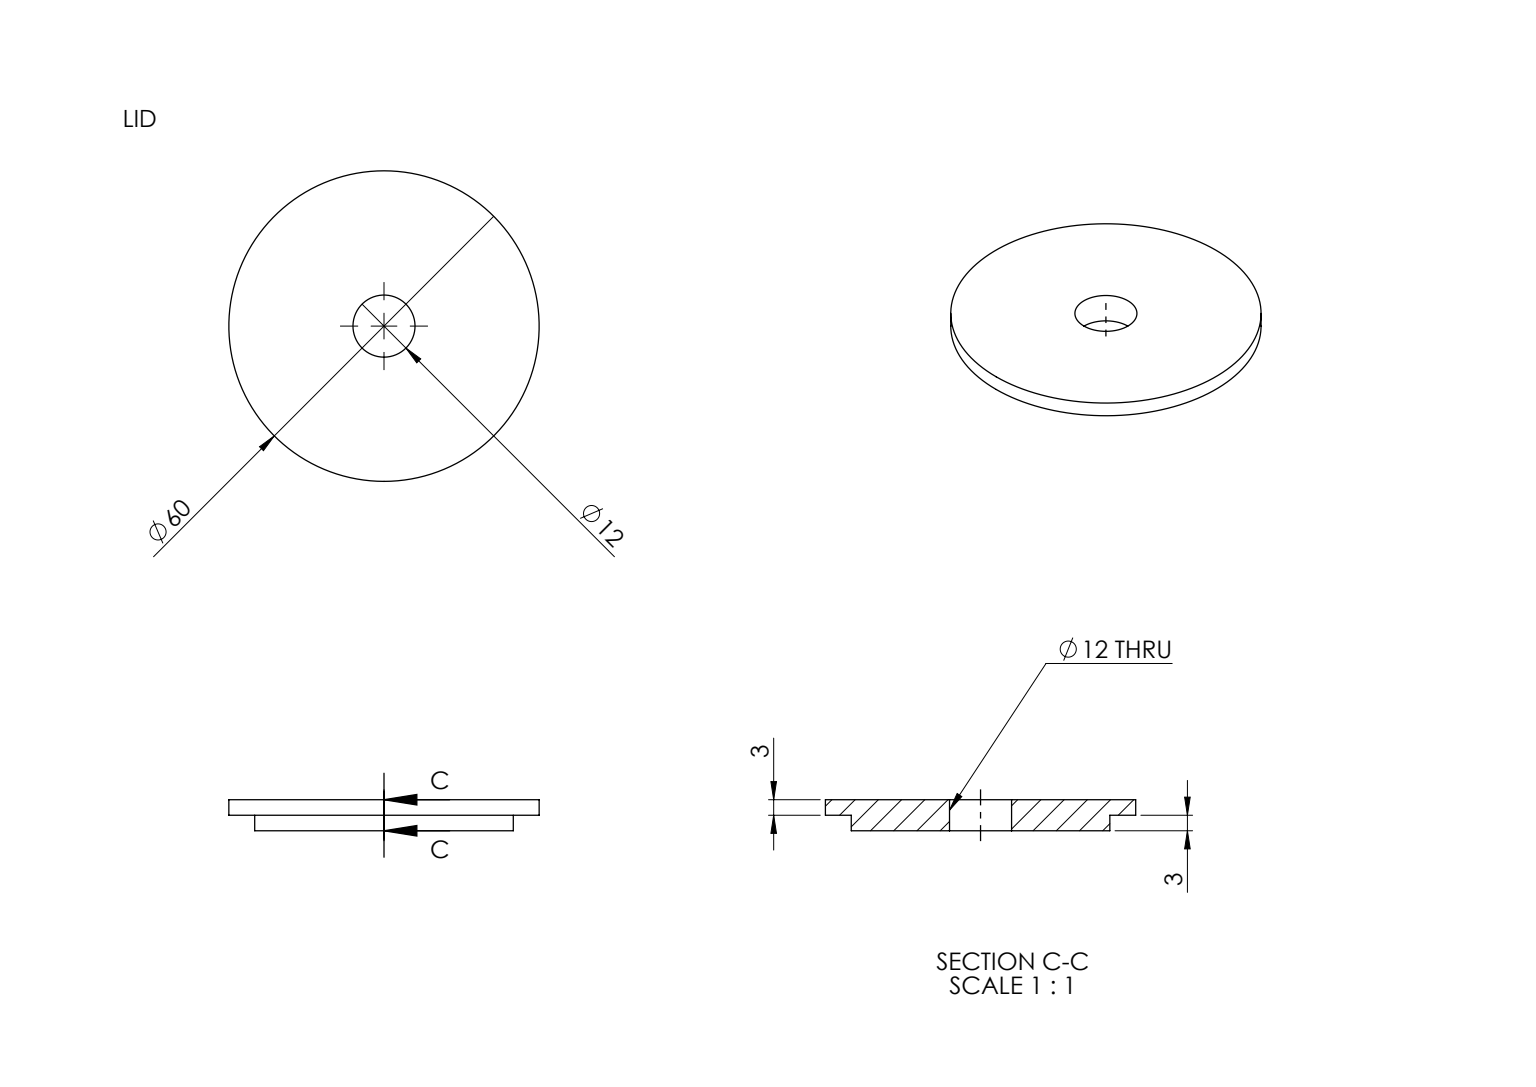
ISO-10303-21;
HEADER;
FILE_DESCRIPTION (('STEP AP214'),
    '1' );
FILE_NAME ('lid.step',
    '2026-10-04T07:23:31',
    ( '' ),
    ( '' ),
    'SwSTEP 2.0',
    'SolidWorks 2026',
    '' );
FILE_SCHEMA (( 'AUTOMOTIVE_DESIGN' ));
ENDSEC;

DATA;
#32=ADVANCED_FACE ( 'NONE', ( #4472 ), #1742, .F. ) ;
#73=CARTESIAN_POINT ( 'NONE',  ( 7.347880794884120722E-16, 82.00000000000000000, -6.000000000000000888 ) ) ;
#113=( NAMED_UNIT ( * ) SI_UNIT ( $, .STERADIAN. ) SOLID_ANGLE_UNIT ( ) );
#161=CARTESIAN_POINT ( 'NONE',  ( 0.000000000000000000, 85.00000000000000000, 0.000000000000000000 ) ) ;
#171=( LENGTH_UNIT ( ) NAMED_UNIT ( * ) SI_UNIT ( .MILLI., .METRE. ) );
#236=VECTOR ( 'NONE', #2762, 1000.000000000000000 ) ;
#246=LINE ( 'NONE', #73, #236 ) ;
#346=VERTEX_POINT ( 'NONE', #9726 ) ;
#355=DIRECTION ( 'NONE',  ( 0.000000000000000000, 1.000000000000000000, 0.000000000000000000 ) ) ;
#357=VECTOR ( 'NONE', #4991, 1000.000000000000000 ) ;
#379=CARTESIAN_POINT ( 'NONE',  ( 0.000000000000000000, 82.00000000000000000, 25.00000000000000000 ) ) ;
#411=FACE_OUTER_BOUND ( 'NONE', #2991, .T. ) ;
#443=EDGE_LOOP ( 'NONE', ( #4090, #2708 ) ) ;
#541=FILL_AREA_STYLE_COLOUR ( '', #3347 ) ;
#542=CARTESIAN_POINT ( 'NONE',  ( 3.061616997868383043E-15, 85.00000000000000000, -25.00000000000000000 ) ) ;
#599=( NAMED_UNIT ( * ) PLANE_ANGLE_UNIT ( ) SI_UNIT ( $, .RADIAN. ) );
#645=EDGE_LOOP ( 'NONE', ( #3984, #3500, #6506, #4878 ) ) ;
#724=LINE ( 'NONE', #5809, #357 ) ;
#759=AXIS2_PLACEMENT_3D ( 'NONE', #1982, #9602, #6241 ) ;
#766=CARTESIAN_POINT ( 'NONE',  ( 0.000000000000000000, 82.00000000000000000, 0.000000000000000000 ) ) ;
#786=CARTESIAN_POINT ( 'NONE',  ( 0.000000000000000000, 82.00000000000000000, 0.000000000000000000 ) ) ;
#791=EDGE_CURVE ( 'NONE', #2046, #346, #7043, .T. ) ;
#911=LINE ( 'NONE', #7643, #8108 ) ;
#959=CYLINDRICAL_SURFACE ( 'NONE', #3390, 6.000000000000000888 ) ;
#1022=DIRECTION ( 'NONE',  ( 0.000000000000000000, 1.000000000000000000, 0.000000000000000000 ) ) ;
#1025=DIRECTION ( 'NONE',  ( 0.000000000000000000, 0.000000000000000000, 1.000000000000000000 ) ) ;
#1035=DIRECTION ( 'NONE',  ( 0.000000000000000000, 1.000000000000000000, 0.000000000000000000 ) ) ;
#1113=FACE_OUTER_BOUND ( 'NONE', #1896, .T. ) ;
#1171=PLANE ( 'NONE',  #8884 ) ;
#1238=CARTESIAN_POINT ( 'NONE',  ( 0.000000000000000000, 82.00000000000000000, 0.000000000000000000 ) ) ;
#1280=( NAMED_UNIT ( * ) SI_UNIT ( $, .STERADIAN. ) SOLID_ANGLE_UNIT ( ) );
#1293=ORIENTED_EDGE ( 'NONE', *, *, #10193, .F. ) ;
#1298=PLANE ( 'NONE',  #6558 ) ;
#1332=PRODUCT ( 'lid', 'lid', '', ( #9152 ) ) ;
#1346=ORIENTED_EDGE ( 'NONE', *, *, #6014, .T. ) ;
#1382=DIRECTION ( 'NONE',  ( 0.000000000000000000, 1.000000000000000000, 0.000000000000000000 ) ) ;
#1465=CIRCLE ( 'NONE', #6577, 30.00000000000000000 ) ;
#1582=DIRECTION ( 'NONE',  ( 0.000000000000000000, 1.000000000000000000, 0.000000000000000000 ) ) ;
#1595=MECHANICAL_DESIGN_GEOMETRIC_PRESENTATION_REPRESENTATION('',(#7787),#10427);
#1619=CIRCLE ( 'NONE', #8151, 6.000000000000000888 ) ;
#1658=VERTEX_POINT ( 'NONE', #7012 ) ;
#1667=DIRECTION ( 'NONE',  ( 0.000000000000000000, 0.000000000000000000, 1.000000000000000000 ) ) ;
#1728=DIRECTION ( 'NONE',  ( 0.000000000000000000, 0.000000000000000000, 1.000000000000000000 ) ) ;
#1742=CYLINDRICAL_SURFACE ( 'NONE', #7907, 6.000000000000000888 ) ;
#1896=EDGE_LOOP ( 'NONE', ( #9721, #7390 ) ) ;
#1904=CARTESIAN_POINT ( 'NONE',  ( 0.000000000000000000, 0.000000000000000000, 0.000000000000000000 ) ) ;
#1945=LINE ( 'NONE', #3530, #6745 ) ;
#1982=CARTESIAN_POINT ( 'NONE',  ( 0.000000000000000000, 85.00000000000000000, 0.000000000000000000 ) ) ;
#2046=VERTEX_POINT ( 'NONE', #3882 ) ;
#2085=AXIS2_PLACEMENT_3D ( 'NONE', #5285, #6996, #1025 ) ;
#2090=ORIENTED_EDGE ( 'NONE', *, *, #10525, .T. ) ;
#2190=CARTESIAN_POINT ( 'NONE',  ( 0.000000000000000000, 88.00000000000001421, 0.000000000000000000 ) ) ;
#2227=ORIENTED_EDGE ( 'NONE', *, *, #4533, .T. ) ;
#2448=DIRECTION ( 'NONE',  ( 0.000000000000000000, -0.000000000000000000, 1.000000000000000000 ) ) ;
#2451=EDGE_CURVE ( 'NONE', #4148, #1658, #724, .T. ) ;
#2496=EDGE_LOOP ( 'NONE', ( #4124, #10919, #4863, #5660 ) ) ;
#2571=EDGE_CURVE ( 'NONE', #2830, #6236, #911, .T. ) ;
#2654=ORIENTED_EDGE ( 'NONE', *, *, #2571, .F. ) ;
#2708=ORIENTED_EDGE ( 'NONE', *, *, #10525, .F. ) ;
#2729=DIRECTION ( 'NONE',  ( 0.000000000000000000, 0.000000000000000000, 1.000000000000000000 ) ) ;
#2762=DIRECTION ( 'NONE',  ( 0.000000000000000000, 1.000000000000000000, 0.000000000000000000 ) ) ;
#2796=CARTESIAN_POINT ( 'NONE',  ( 0.000000000000000000, 85.00000000000000000, 0.000000000000000000 ) ) ;
#2821=CARTESIAN_POINT ( 'NONE',  ( 0.000000000000000000, 88.00000000000001421, 0.000000000000000000 ) ) ;
#2830=VERTEX_POINT ( 'NONE', #9435 ) ;
#2833=VECTOR ( 'NONE', #4440, 1000.000000000000000 ) ;
#2964=ORIENTED_EDGE ( 'NONE', *, *, #7197, .T. ) ;
#2984=EDGE_CURVE ( 'NONE', #6236, #1658, #4434, .T. ) ;
#2991=EDGE_LOOP ( 'NONE', ( #6706, #7409 ) ) ;
#3041=UNCERTAINTY_MEASURE_WITH_UNIT (LENGTH_MEASURE( 1.000000000000000082E-05 ), #5577, 'distance_accuracy_value', 'NONE');
#3072=SURFACE_STYLE_FILL_AREA ( #5529 ) ;
#3103=FACE_OUTER_BOUND ( 'NONE', #5298, .T. ) ;
#3222=SURFACE_SIDE_STYLE ('',( #10822 ) ) ;
#3230=VERTEX_POINT ( 'NONE', #10545 ) ;
#3247=EDGE_CURVE ( 'NONE', #7302, #6283, #9549, .T. ) ;
#3256=FACE_OUTER_BOUND ( 'NONE', #2496, .T. ) ;
#3276=DIRECTION ( 'NONE',  ( 0.000000000000000000, 0.000000000000000000, 1.000000000000000000 ) ) ;
#3290=CARTESIAN_POINT ( 'NONE',  ( 0.000000000000000000, 85.00000000000000000, 0.000000000000000000 ) ) ;
#3337=AXIS2_PLACEMENT_3D ( 'NONE', #3290, #1382, #4824 ) ;
#3347=COLOUR_RGB ( '', 0.66274510, 0.83137255, 0.94901961) ;
#3360=MANIFOLD_SOLID_BREP ( 'Boss-Extrude2', #5953 ) ;
#3390=AXIS2_PLACEMENT_3D ( 'NONE', #786, #7684, #1667 ) ;
#3428=DIRECTION ( 'NONE',  ( 0.000000000000000000, 1.000000000000000000, 0.000000000000000000 ) ) ;
#3431=DIRECTION ( 'NONE',  ( 0.000000000000000000, 0.000000000000000000, 1.000000000000000000 ) ) ;
#3473=CARTESIAN_POINT ( 'NONE',  ( 0.000000000000000000, 88.00000000000001421, 0.000000000000000000 ) ) ;
#3500=ORIENTED_EDGE ( 'NONE', *, *, #6344, .T. ) ;
#3503=ORIENTED_EDGE ( 'NONE', *, *, #3247, .F. ) ;
#3530=CARTESIAN_POINT ( 'NONE',  ( 3.061616997868383043E-15, 82.00000000000000000, -25.00000000000000000 ) ) ;
#3709=SURFACE_SIDE_STYLE ('',( #3072 ) ) ;
#3757=EDGE_CURVE ( 'NONE', #3230, #4608, #10227, .T. ) ;
#3793=CARTESIAN_POINT ( 'NONE',  ( 0.000000000000000000, 85.00000000000000000, 0.000000000000000000 ) ) ;
#3812=SURFACE_STYLE_USAGE ( .BOTH. , #3709 ) ;
#3882=CARTESIAN_POINT ( 'NONE',  ( 3.061616997868383043E-15, 82.00000000000000000, -25.00000000000000000 ) ) ;
#3888=ORIENTED_EDGE ( 'NONE', *, *, #10193, .T. ) ;
#3903=EDGE_CURVE ( 'NONE', #6283, #3230, #5920, .T. ) ;
#3953=UNCERTAINTY_MEASURE_WITH_UNIT (LENGTH_MEASURE( 1.000000000000000082E-05 ), #171, 'distance_accuracy_value', 'NONE');
#3961=VERTEX_POINT ( 'NONE', #7229 ) ;
#3984=ORIENTED_EDGE ( 'NONE', *, *, #10172, .T. ) ;
#4082=AXIS2_PLACEMENT_3D ( 'NONE', #9184, #9905, #4952 ) ;
#4090=ORIENTED_EDGE ( 'NONE', *, *, #3757, .F. ) ;
#4113=CIRCLE ( 'NONE', #5518, 25.00000000000000000 ) ;
#4124=ORIENTED_EDGE ( 'NONE', *, *, #6344, .F. ) ;
#4125=AXIS2_PLACEMENT_3D ( 'NONE', #6667, #10026, #2448 ) ;
#4131=AXIS2_PLACEMENT_3D ( 'NONE', #3793, #7165, #2729 ) ;
#4132=FACE_BOUND ( 'NONE', #443, .T. ) ;
#4148=VERTEX_POINT ( 'NONE', #6512 ) ;
#4155=DIRECTION ( 'NONE',  ( 0.000000000000000000, 1.000000000000000000, 0.000000000000000000 ) ) ;
#4204=FACE_OUTER_BOUND ( 'NONE', #4707, .T. ) ;
#4368=MECHANICAL_DESIGN_GEOMETRIC_PRESENTATION_REPRESENTATION('',(#10889),#10535);
#4418=PRODUCT_DEFINITION_FORMATION_WITH_SPECIFIED_SOURCE ( 'ANY', '', #1332, .NOT_KNOWN. ) ;
#4434=CIRCLE ( 'NONE', #3337, 30.00000000000000000 ) ;
#4440=DIRECTION ( 'NONE',  ( 0.000000000000000000, 1.000000000000000000, 0.000000000000000000 ) ) ;
#4472=FACE_OUTER_BOUND ( 'NONE', #10773, .T. ) ;
#4496=DIRECTION ( 'NONE',  ( 0.000000000000000000, 1.000000000000000000, 0.000000000000000000 ) ) ;
#4533=EDGE_CURVE ( 'NONE', #3961, #10543, #9708, .T. ) ;
#4572=DIRECTION ( 'NONE',  ( 0.000000000000000000, 0.000000000000000000, 1.000000000000000000 ) ) ;
#4585=FACE_OUTER_BOUND ( 'NONE', #9652, .T. ) ;
#4608=VERTEX_POINT ( 'NONE', #9501 ) ;
#4645=DIRECTION ( 'NONE',  ( 0.000000000000000000, 1.000000000000000000, 0.000000000000000000 ) ) ;
#4662=PRESENTATION_STYLE_ASSIGNMENT (( #3812 ) ) ;
#4707=EDGE_LOOP ( 'NONE', ( #3503, #3888, #2090, #5456 ) ) ;
#4779=ORIENTED_EDGE ( 'NONE', *, *, #2571, .T. ) ;
#4824=DIRECTION ( 'NONE',  ( 0.000000000000000000, 0.000000000000000000, 1.000000000000000000 ) ) ;
#4863=ORIENTED_EDGE ( 'NONE', *, *, #7668, .T. ) ;
#4878=ORIENTED_EDGE ( 'NONE', *, *, #7668, .F. ) ;
#4905=ADVANCED_FACE ( 'NONE', ( #9430, #4132 ), #8592, .T. ) ;
#4916=SHAPE_DEFINITION_REPRESENTATION ( #6369, #7685 ) ;
#4952=DIRECTION ( 'NONE',  ( 0.000000000000000000, 0.000000000000000000, 1.000000000000000000 ) ) ;
#4991=DIRECTION ( 'NONE',  ( -0.000000000000000000, -1.000000000000000000, -0.000000000000000000 ) ) ;
#5007=ADVANCED_FACE ( 'NONE', ( #4585 ), #6960, .T. ) ;
#5022=AXIS2_PLACEMENT_3D ( 'NONE', #7933, #9542, #8809 ) ;
#5051=EDGE_CURVE ( 'NONE', #10543, #3961, #10831, .T. ) ;
#5063=CYLINDRICAL_SURFACE ( 'NONE', #4082, 25.00000000000000000 ) ;
#5104=DIRECTION ( 'NONE',  ( 0.000000000000000000, 0.000000000000000000, 1.000000000000000000 ) ) ;
#5152=CARTESIAN_POINT ( 'NONE',  ( 0.000000000000000000, 85.00000000000000000, -30.00000000000000000 ) ) ;
#5285=CARTESIAN_POINT ( 'NONE',  ( 0.000000000000000000, 82.00000000000000000, 0.000000000000000000 ) ) ;
#5298=EDGE_LOOP ( 'NONE', ( #10761, #10694, #1346, #2654 ) ) ;
#5372=DIRECTION ( 'NONE',  ( 0.000000000000000000, 1.000000000000000000, 0.000000000000000000 ) ) ;
#5417=FACE_BOUND ( 'NONE', #5943, .T. ) ;
#5421=ORIENTED_EDGE ( 'NONE', *, *, #3757, .T. ) ;
#5440=FACE_BOUND ( 'NONE', #8351, .T. ) ;
#5456=ORIENTED_EDGE ( 'NONE', *, *, #3903, .F. ) ;
#5518=AXIS2_PLACEMENT_3D ( 'NONE', #7814, #1022, #1728 ) ;
#5529=FILL_AREA_STYLE ('',( #10550 ) ) ;
#5548=DIRECTION ( 'NONE',  ( 0.000000000000000000, 1.000000000000000000, 0.000000000000000000 ) ) ;
#5568=DIRECTION ( 'NONE',  ( -0.000000000000000000, -1.000000000000000000, -0.000000000000000000 ) ) ;
#5577=( LENGTH_UNIT ( ) NAMED_UNIT ( * ) SI_UNIT ( .MILLI., .METRE. ) );
#5653=DIRECTION ( 'NONE',  ( 0.000000000000000000, -0.000000000000000000, 1.000000000000000000 ) ) ;
#5660=ORIENTED_EDGE ( 'NONE', *, *, #5051, .F. ) ;
#5675=CYLINDRICAL_SURFACE ( 'NONE', #8858, 30.00000000000000000 ) ;
#5809=CARTESIAN_POINT ( 'NONE',  ( 3.673940397442059178E-15, 88.00000000000001421, 30.00000000000000000 ) ) ;
#5876=ORIENTED_EDGE ( 'NONE', *, *, #10242, .T. ) ;
#5877=CIRCLE ( 'NONE', #8705, 30.00000000000000000 ) ;
#5920=LINE ( 'NONE', #8621, #2833 ) ;
#5943=EDGE_LOOP ( 'NONE', ( #2227, #10087 ) ) ;
#5953=CLOSED_SHELL ( 'NONE', ( #6598, #7172, #10910, #8544, #8762, #32, #4905, #7690, #5007 ) ) ;
#5967=ORIENTED_EDGE ( 'NONE', *, *, #2451, .F. ) ;
#6014=EDGE_CURVE ( 'NONE', #1658, #6236, #10302, .T. ) ;
#6236=VERTEX_POINT ( 'NONE', #5152 ) ;
#6241=DIRECTION ( 'NONE',  ( 0.000000000000000000, 0.000000000000000000, 1.000000000000000000 ) ) ;
#6283=VERTEX_POINT ( 'NONE', #7799 ) ;
#6308=COLOUR_RGB ( '', 0.66274510, 0.83137255, 0.94901961) ;
#6344=EDGE_CURVE ( 'NONE', #2046, #10543, #1945, .T. ) ;
#6369=PRODUCT_DEFINITION_SHAPE ( 'NONE', 'NONE',  #8124 ) ;
#6411=EDGE_CURVE ( 'NONE', #6283, #7302, #1619, .T. ) ;
#6432=EDGE_LOOP ( 'NONE', ( #2964, #5876 ) ) ;
#6506=ORIENTED_EDGE ( 'NONE', *, *, #4533, .F. ) ;
#6512=CARTESIAN_POINT ( 'NONE',  ( 3.673940397442059178E-15, 88.00000000000001421, 30.00000000000000000 ) ) ;
#6558=AXIS2_PLACEMENT_3D ( 'NONE', #7155, #355, #5653 ) ;
#6577=AXIS2_PLACEMENT_3D ( 'NONE', #3473, #4155, #8345 ) ;
#6598=ADVANCED_FACE ( 'NONE', ( #3103 ), #5675, .T. ) ;
#6619=SURFACE_STYLE_USAGE ( .BOTH. , #3222 ) ;
#6667=CARTESIAN_POINT ( 'NONE',  ( 0.000000000000000000, 88.00000000000001421, 0.000000000000000000 ) ) ;
#6706=ORIENTED_EDGE ( 'NONE', *, *, #10172, .F. ) ;
#6745=VECTOR ( 'NONE', #9512, 1000.000000000000000 ) ;
#6893=DIRECTION ( 'NONE',  ( 0.000000000000000000, 0.000000000000000000, 1.000000000000000000 ) ) ;
#6908=ORIENTED_EDGE ( 'NONE', *, *, #6411, .F. ) ;
#6960=CYLINDRICAL_SURFACE ( 'NONE', #5022, 30.00000000000000000 ) ;
#6996=DIRECTION ( 'NONE',  ( 0.000000000000000000, 1.000000000000000000, 0.000000000000000000 ) ) ;
#7012=CARTESIAN_POINT ( 'NONE',  ( 3.673940397442059178E-15, 85.00000000000000000, 30.00000000000000000 ) ) ;
#7026=( GEOMETRIC_REPRESENTATION_CONTEXT ( 3 ) GLOBAL_UNCERTAINTY_ASSIGNED_CONTEXT ( ( #3953 ) ) GLOBAL_UNIT_ASSIGNED_CONTEXT ( ( #171, #9327, #113 ) ) REPRESENTATION_CONTEXT ( 'NONE', 'WORKASPACE' ) );
#7040=AXIS2_PLACEMENT_3D ( 'NONE', #1904, #3431, #7048 ) ;
#7043=CIRCLE ( 'NONE', #8242, 25.00000000000000000 ) ;
#7048=DIRECTION ( 'NONE',  ( 1.000000000000000000, 0.000000000000000000, 0.000000000000000000 ) ) ;
#7137=DIRECTION ( 'NONE',  ( 0.000000000000000000, 0.000000000000000000, 1.000000000000000000 ) ) ;
#7155=CARTESIAN_POINT ( 'NONE',  ( 0.000000000000000000, 82.00000000000000000, 0.000000000000000000 ) ) ;
#7165=DIRECTION ( 'NONE',  ( 0.000000000000000000, 1.000000000000000000, 0.000000000000000000 ) ) ;
#7172=ADVANCED_FACE ( 'NONE', ( #4204 ), #959, .F. ) ;
#7185=( NAMED_UNIT ( * ) PLANE_ANGLE_UNIT ( ) SI_UNIT ( $, .RADIAN. ) );
#7186=CARTESIAN_POINT ( 'NONE',  ( 7.347880794884120722E-16, 82.00000000000000000, -6.000000000000000888 ) ) ;
#7197=EDGE_CURVE ( 'NONE', #2830, #4148, #1465, .T. ) ;
#7229=CARTESIAN_POINT ( 'NONE',  ( 0.000000000000000000, 85.00000000000000000, 25.00000000000000000 ) ) ;
#7278=( NAMED_UNIT ( * ) SI_UNIT ( $, .STERADIAN. ) SOLID_ANGLE_UNIT ( ) );
#7298=DIRECTION ( 'NONE',  ( 0.000000000000000000, 1.000000000000000000, 0.000000000000000000 ) ) ;
#7302=VERTEX_POINT ( 'NONE', #7186 ) ;
#7316=DIRECTION ( 'NONE',  ( 0.000000000000000000, 0.000000000000000000, -1.000000000000000000 ) ) ;
#7390=ORIENTED_EDGE ( 'NONE', *, *, #6014, .F. ) ;
#7399=DIRECTION ( 'NONE',  ( 0.000000000000000000, 0.000000000000000000, 1.000000000000000000 ) ) ;
#7409=ORIENTED_EDGE ( 'NONE', *, *, #791, .F. ) ;
#7418=DIRECTION ( 'NONE',  ( -0.000000000000000000, -1.000000000000000000, -0.000000000000000000 ) ) ;
#7435=DIRECTION ( 'NONE',  ( 0.000000000000000000, 0.000000000000000000, 1.000000000000000000 ) ) ;
#7470=ORIENTED_EDGE ( 'NONE', *, *, #3247, .T. ) ;
#7499=CARTESIAN_POINT ( 'NONE',  ( 0.000000000000000000, 88.00000000000001421, 0.000000000000000000 ) ) ;
#7504=LINE ( 'NONE', #379, #7834 ) ;
#7538=CIRCLE ( 'NONE', #10003, 6.000000000000000888 ) ;
#7643=CARTESIAN_POINT ( 'NONE',  ( 0.000000000000000000, 88.00000000000001421, -30.00000000000000000 ) ) ;
#7652=CARTESIAN_POINT ( 'NONE',  ( 0.000000000000000000, 82.00000000000000000, 0.000000000000000000 ) ) ;
#7668=EDGE_CURVE ( 'NONE', #346, #3961, #7504, .T. ) ;
#7684=DIRECTION ( 'NONE',  ( 0.000000000000000000, 1.000000000000000000, 0.000000000000000000 ) ) ;
#7685=SHAPE_REPRESENTATION ( 'lid', ( #7040 ), #7026 ) ;
#7690=ADVANCED_FACE ( 'NONE', ( #5417, #1113 ), #1171, .F. ) ;
#7771=AXIS2_PLACEMENT_3D ( 'NONE', #2796, #4645, #10435 ) ;
#7787=STYLED_ITEM ( 'NONE', ( #10600 ), #3360 ) ;
#7799=CARTESIAN_POINT ( 'NONE',  ( 0.000000000000000000, 82.00000000000000000, 6.000000000000000888 ) ) ;
#7814=CARTESIAN_POINT ( 'NONE',  ( 0.000000000000000000, 82.00000000000000000, 0.000000000000000000 ) ) ;
#7834=VECTOR ( 'NONE', #4496, 1000.000000000000000 ) ;
#7907=AXIS2_PLACEMENT_3D ( 'NONE', #7652, #1035, #6893 ) ;
#7933=CARTESIAN_POINT ( 'NONE',  ( 0.000000000000000000, 88.00000000000001421, 0.000000000000000000 ) ) ;
#8108=VECTOR ( 'NONE', #7418, 1000.000000000000000 ) ;
#8124=PRODUCT_DEFINITION ( 'UNKNOWN', '', #4418, #9123 ) ;
#8151=AXIS2_PLACEMENT_3D ( 'NONE', #766, #1582, #7435 ) ;
#8167=FILL_AREA_STYLE ('',( #541 ) ) ;
#8242=AXIS2_PLACEMENT_3D ( 'NONE', #1238, #5548, #4572 ) ;
#8345=DIRECTION ( 'NONE',  ( 0.000000000000000000, 0.000000000000000000, 1.000000000000000000 ) ) ;
#8351=EDGE_LOOP ( 'NONE', ( #8454, #7470 ) ) ;
#8369=ORIENTED_EDGE ( 'NONE', *, *, #3903, .T. ) ;
#8454=ORIENTED_EDGE ( 'NONE', *, *, #6411, .T. ) ;
#8544=ADVANCED_FACE ( 'NONE', ( #3256 ), #5063, .T. ) ;
#8592=PLANE ( 'NONE',  #4125 ) ;
#8621=CARTESIAN_POINT ( 'NONE',  ( 0.000000000000000000, 82.00000000000000000, 6.000000000000000888 ) ) ;
#8675=CARTESIAN_POINT ( 'NONE',  ( 0.000000000000000000, 82.00000000000000000, 0.000000000000000000 ) ) ;
#8705=AXIS2_PLACEMENT_3D ( 'NONE', #2821, #3428, #5104 ) ;
#8752=FACE_OUTER_BOUND ( 'NONE', #645, .T. ) ;
#8762=ADVANCED_FACE ( 'NONE', ( #5440, #411 ), #1298, .F. ) ;
#8787=SHAPE_REPRESENTATION_RELATIONSHIP ( 'NONE' , 'NONE' ,  #7685, #9142 ) ;
#8794=APPLICATION_CONTEXT ( 'automotive_design' ) ;
#8809=DIRECTION ( 'NONE',  ( 0.000000000000000000, 0.000000000000000000, -1.000000000000000000 ) ) ;
#8823=DIRECTION ( 'NONE',  ( 0.000000000000000000, -0.000000000000000000, 1.000000000000000000 ) ) ;
#8858=AXIS2_PLACEMENT_3D ( 'NONE', #2190, #5568, #7316 ) ;
#8884=AXIS2_PLACEMENT_3D ( 'NONE', #161, #5372, #8823 ) ;
#9033=ORIENTED_EDGE ( 'NONE', *, *, #2984, .T. ) ;
#9123=PRODUCT_DEFINITION_CONTEXT ( 'detailed design', #8794, 'design' ) ;
#9142=ADVANCED_BREP_SHAPE_REPRESENTATION ( '', ( #3360, #7040 ), #7026 ) ;
#9152=PRODUCT_CONTEXT ( 'NONE', #9576, 'mechanical' ) ;
#9184=CARTESIAN_POINT ( 'NONE',  ( 0.000000000000000000, 82.00000000000000000, 0.000000000000000000 ) ) ;
#9327=( NAMED_UNIT ( * ) PLANE_ANGLE_UNIT ( ) SI_UNIT ( $, .RADIAN. ) );
#9430=FACE_OUTER_BOUND ( 'NONE', #6432, .T. ) ;
#9435=CARTESIAN_POINT ( 'NONE',  ( 0.000000000000000000, 88.00000000000001421, -30.00000000000000000 ) ) ;
#9501=CARTESIAN_POINT ( 'NONE',  ( 7.347880794884120722E-16, 88.00000000000001421, -6.000000000000000888 ) ) ;
#9512=DIRECTION ( 'NONE',  ( 0.000000000000000000, 1.000000000000000000, 0.000000000000000000 ) ) ;
#9528=CYLINDRICAL_SURFACE ( 'NONE', #2085, 25.00000000000000000 ) ;
#9542=DIRECTION ( 'NONE',  ( -0.000000000000000000, -1.000000000000000000, -0.000000000000000000 ) ) ;
#9549=CIRCLE ( 'NONE', #10943, 6.000000000000000888 ) ;
#9576=APPLICATION_CONTEXT ( 'automotive_design' ) ;
#9602=DIRECTION ( 'NONE',  ( 0.000000000000000000, 1.000000000000000000, 0.000000000000000000 ) ) ;
#9652=EDGE_LOOP ( 'NONE', ( #5967, #10041, #4779, #9033 ) ) ;
#9708=CIRCLE ( 'NONE', #7771, 25.00000000000000000 ) ;
#9721=ORIENTED_EDGE ( 'NONE', *, *, #2984, .F. ) ;
#9726=CARTESIAN_POINT ( 'NONE',  ( 0.000000000000000000, 82.00000000000000000, 25.00000000000000000 ) ) ;
#9886=AXIS2_PLACEMENT_3D ( 'NONE', #9944, #7298, #7399 ) ;
#9905=DIRECTION ( 'NONE',  ( 0.000000000000000000, 1.000000000000000000, 0.000000000000000000 ) ) ;
#9944=CARTESIAN_POINT ( 'NONE',  ( 0.000000000000000000, 88.00000000000001421, 0.000000000000000000 ) ) ;
#10003=AXIS2_PLACEMENT_3D ( 'NONE', #7499, #10877, #3276 ) ;
#10026=DIRECTION ( 'NONE',  ( 0.000000000000000000, 1.000000000000000000, 0.000000000000000000 ) ) ;
#10041=ORIENTED_EDGE ( 'NONE', *, *, #7197, .F. ) ;
#10087=ORIENTED_EDGE ( 'NONE', *, *, #5051, .T. ) ;
#10172=EDGE_CURVE ( 'NONE', #346, #2046, #4113, .T. ) ;
#10193=EDGE_CURVE ( 'NONE', #7302, #4608, #246, .T. ) ;
#10227=CIRCLE ( 'NONE', #9886, 6.000000000000000888 ) ;
#10242=EDGE_CURVE ( 'NONE', #4148, #2830, #5877, .T. ) ;
#10302=CIRCLE ( 'NONE', #759, 30.00000000000000000 ) ;
#10337=DIRECTION ( 'NONE',  ( 0.000000000000000000, 1.000000000000000000, 0.000000000000000000 ) ) ;
#10427=( GEOMETRIC_REPRESENTATION_CONTEXT ( 3 ) GLOBAL_UNCERTAINTY_ASSIGNED_CONTEXT ( ( #3041 ) ) GLOBAL_UNIT_ASSIGNED_CONTEXT ( ( #5577, #599, #7278 ) ) REPRESENTATION_CONTEXT ( 'NONE', 'WORKASPACE' ) );
#10435=DIRECTION ( 'NONE',  ( 0.000000000000000000, 0.000000000000000000, 1.000000000000000000 ) ) ;
#10525=EDGE_CURVE ( 'NONE', #4608, #3230, #7538, .T. ) ;
#10535=( GEOMETRIC_REPRESENTATION_CONTEXT ( 3 ) GLOBAL_UNCERTAINTY_ASSIGNED_CONTEXT ( ( #10683 ) ) GLOBAL_UNIT_ASSIGNED_CONTEXT ( ( #10605, #7185, #1280 ) ) REPRESENTATION_CONTEXT ( 'NONE', 'WORKASPACE' ) );
#10543=VERTEX_POINT ( 'NONE', #542 ) ;
#10545=CARTESIAN_POINT ( 'NONE',  ( 0.000000000000000000, 88.00000000000001421, 6.000000000000000888 ) ) ;
#10550=FILL_AREA_STYLE_COLOUR ( '', #6308 ) ;
#10600=PRESENTATION_STYLE_ASSIGNMENT (( #6619 ) ) ;
#10605=( LENGTH_UNIT ( ) NAMED_UNIT ( * ) SI_UNIT ( .MILLI., .METRE. ) );
#10683=UNCERTAINTY_MEASURE_WITH_UNIT (LENGTH_MEASURE( 1.000000000000000082E-05 ), #10605, 'distance_accuracy_value', 'NONE');
#10694=ORIENTED_EDGE ( 'NONE', *, *, #2451, .T. ) ;
#10761=ORIENTED_EDGE ( 'NONE', *, *, #10242, .F. ) ;
#10773=EDGE_LOOP ( 'NONE', ( #1293, #6908, #8369, #5421 ) ) ;
#10822=SURFACE_STYLE_FILL_AREA ( #8167 ) ;
#10831=CIRCLE ( 'NONE', #4131, 25.00000000000000000 ) ;
#10877=DIRECTION ( 'NONE',  ( 0.000000000000000000, 1.000000000000000000, 0.000000000000000000 ) ) ;
#10889=STYLED_ITEM ( 'NONE', ( #4662 ), #9142 ) ;
#10910=ADVANCED_FACE ( 'NONE', ( #8752 ), #9528, .T. ) ;
#10919=ORIENTED_EDGE ( 'NONE', *, *, #791, .T. ) ;
#10943=AXIS2_PLACEMENT_3D ( 'NONE', #8675, #10337, #7137 ) ;
ENDSEC;
END-ISO-10303-21;
